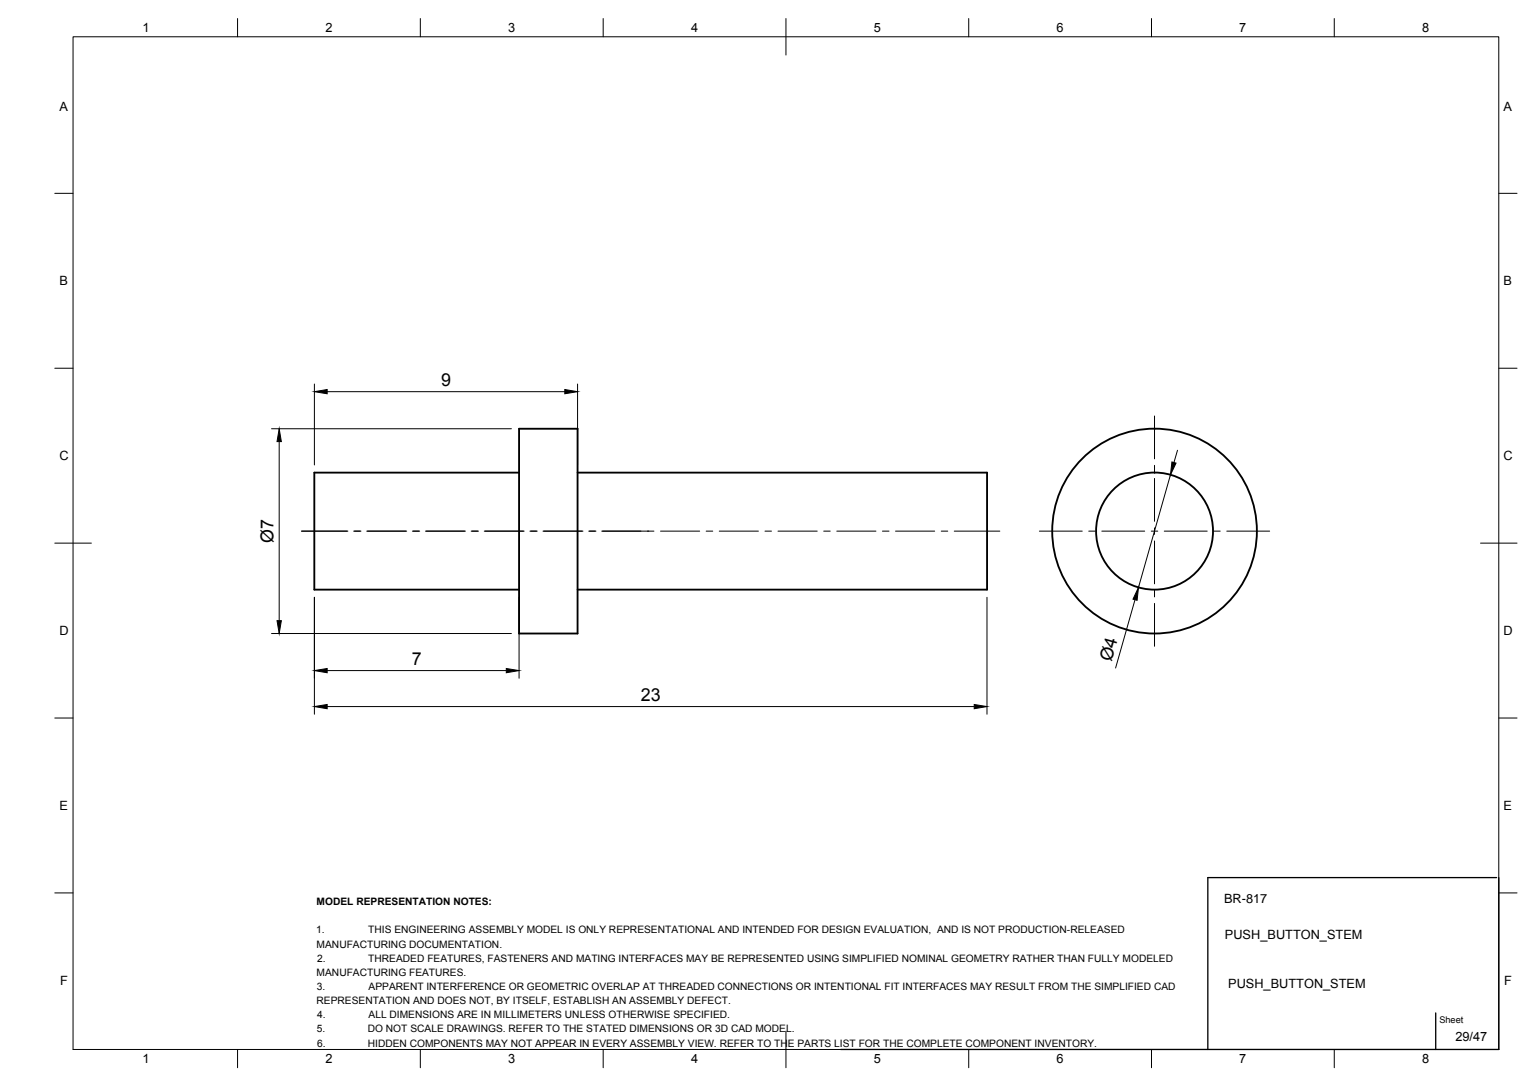
ISO-10303-21;
HEADER;
FILE_DESCRIPTION((''),'2;1');
FILE_NAME('PUSH_BUTTON_STEM.step','2026-10-01T22:07:29-07:00',(''),(''),'','','');
FILE_SCHEMA (('AUTOMOTIVE_DESIGN { 1 0 10303 214 3 1 1 }'));
ENDSEC;
DATA;
#10=MECHANICAL_DESIGN_GEOMETRIC_PRESENTATION_REPRESENTATION('',(#561),#15484);
#491=SHAPE_REPRESENTATION_RELATIONSHIP('SRR','None',#15641,#526) ;
#526=ADVANCED_BREP_SHAPE_REPRESENTATION('',(#602),#15465) ;
#561=STYLED_ITEM('',(#15833),#602) ;
#602=MANIFOLD_SOLID_BREP('PUSH_BUTTON_STEM',#8272) ;
#728=CYLINDRICAL_SURFACE('',#9326,0.35) ;
#729=CYLINDRICAL_SURFACE('',#9327,0.2) ;
#730=CYLINDRICAL_SURFACE('',#9329,0.2) ;
#871=FACE_BOUND('',#2197,.T.) ;
#872=FACE_BOUND('',#2199,.T.) ;
#1139=CIRCLE('',#9321,0.35) ;
#1140=CIRCLE('',#9322,0.2) ;
#1141=CIRCLE('',#9324,0.35) ;
#1142=CIRCLE('',#9325,0.2) ;
#1143=CIRCLE('',#9328,0.2) ;
#1144=CIRCLE('',#9330,0.2) ;
#1635=FACE_OUTER_BOUND('',#2196,.T.) ;
#1636=FACE_OUTER_BOUND('',#2198,.T.) ;
#1637=FACE_OUTER_BOUND('',#2200,.T.) ;
#1638=FACE_OUTER_BOUND('',#2201,.T.) ;
#1639=FACE_OUTER_BOUND('',#2202,.T.) ;
#1640=FACE_OUTER_BOUND('',#2203,.T.) ;
#1641=FACE_OUTER_BOUND('',#2204,.T.) ;
#2196=EDGE_LOOP('',(#6493)) ;
#2197=EDGE_LOOP('',(#6494)) ;
#2198=EDGE_LOOP('',(#6495)) ;
#2199=EDGE_LOOP('',(#6496)) ;
#2200=EDGE_LOOP('',(#6497,#6498,#6499,#6500)) ;
#2201=EDGE_LOOP('',(#6501,#6502,#6503,#6504)) ;
#2202=EDGE_LOOP('',(#6505,#6506,#6507,#6508)) ;
#2203=EDGE_LOOP('',(#6509)) ;
#2204=EDGE_LOOP('',(#6510)) ;
#2719=LINE('',#14264,#3193) ;
#2720=LINE('',#14268,#3194) ;
#2721=LINE('',#14271,#3195) ;
#3193=VECTOR('',#11494,0.35) ;
#3194=VECTOR('',#11499,0.2) ;
#3195=VECTOR('',#11502,0.2) ;
#3795=VERTEX_POINT('',#14254) ;
#3796=VERTEX_POINT('',#14256) ;
#3797=VERTEX_POINT('',#14259) ;
#3798=VERTEX_POINT('',#14261) ;
#3799=VERTEX_POINT('',#14266) ;
#3800=VERTEX_POINT('',#14270) ;
#4751=EDGE_CURVE('',#3795,#3795,#1139,.T.) ;
#4752=EDGE_CURVE('',#3796,#3796,#1140,.T.) ;
#4753=EDGE_CURVE('',#3797,#3797,#1141,.T.) ;
#4754=EDGE_CURVE('',#3798,#3798,#1142,.T.) ;
#4755=EDGE_CURVE('',#3797,#3795,#2719,.T.) ;
#4756=EDGE_CURVE('',#3799,#3799,#1143,.T.) ;
#4757=EDGE_CURVE('',#3799,#3798,#2720,.T.) ;
#4758=EDGE_CURVE('',#3796,#3800,#2721,.T.) ;
#4759=EDGE_CURVE('',#3800,#3800,#1144,.T.) ;
#6493=ORIENTED_EDGE('',*,*,#4751,.T.) ;
#6494=ORIENTED_EDGE('',*,*,#4752,.F.) ;
#6495=ORIENTED_EDGE('',*,*,#4753,.T.) ;
#6496=ORIENTED_EDGE('',*,*,#4754,.F.) ;
#6497=ORIENTED_EDGE('',*,*,#4753,.F.) ;
#6498=ORIENTED_EDGE('',*,*,#4755,.T.) ;
#6499=ORIENTED_EDGE('',*,*,#4751,.F.) ;
#6500=ORIENTED_EDGE('',*,*,#4755,.F.) ;
#6501=ORIENTED_EDGE('',*,*,#4756,.F.) ;
#6502=ORIENTED_EDGE('',*,*,#4757,.T.) ;
#6503=ORIENTED_EDGE('',*,*,#4754,.T.) ;
#6504=ORIENTED_EDGE('',*,*,#4757,.F.) ;
#6505=ORIENTED_EDGE('',*,*,#4752,.T.) ;
#6506=ORIENTED_EDGE('',*,*,#4758,.T.) ;
#6507=ORIENTED_EDGE('',*,*,#4759,.F.) ;
#6508=ORIENTED_EDGE('',*,*,#4758,.F.) ;
#6509=ORIENTED_EDGE('',*,*,#4759,.T.) ;
#6510=ORIENTED_EDGE('',*,*,#4756,.T.) ;
#7660=PLANE('',#9320) ;
#7661=PLANE('',#9323) ;
#7662=PLANE('',#9331) ;
#7663=PLANE('',#9332) ;
#8022=ADVANCED_FACE('',(#1635,#871),#7660,.T.) ;
#8023=ADVANCED_FACE('',(#1636,#872),#7661,.T.) ;
#8024=ADVANCED_FACE('',(#1637),#728,.T.) ;
#8025=ADVANCED_FACE('',(#1638),#729,.T.) ;
#8026=ADVANCED_FACE('',(#1639),#730,.T.) ;
#8027=ADVANCED_FACE('',(#1640),#7662,.T.) ;
#8028=ADVANCED_FACE('',(#1641),#7663,.T.) ;
#8272=CLOSED_SHELL('',(#8022,#8023,#8024,#8025,#8026,#8027,#8028)) ;
#9319=AXIS2_PLACEMENT_3D('',#14252,#11478,#11479) ;
#9320=AXIS2_PLACEMENT_3D('',#14253,#11480,#11481) ;
#9321=AXIS2_PLACEMENT_3D('',#14255,#11482,#11483) ;
#9322=AXIS2_PLACEMENT_3D('',#14257,#11484,#11485) ;
#9323=AXIS2_PLACEMENT_3D('',#14258,#11486,#11487) ;
#9324=AXIS2_PLACEMENT_3D('',#14260,#11488,#11489) ;
#9325=AXIS2_PLACEMENT_3D('',#14262,#11490,#11491) ;
#9326=AXIS2_PLACEMENT_3D('',#14263,#11492,#11493) ;
#9327=AXIS2_PLACEMENT_3D('',#14265,#11495,#11496) ;
#9328=AXIS2_PLACEMENT_3D('',#14267,#11497,#11498) ;
#9329=AXIS2_PLACEMENT_3D('',#14269,#11500,#11501) ;
#9330=AXIS2_PLACEMENT_3D('',#14272,#11503,#11504) ;
#9331=AXIS2_PLACEMENT_3D('',#14273,#11505,#11506) ;
#9332=AXIS2_PLACEMENT_3D('',#14274,#11507,#11508) ;
#11478=DIRECTION('axis',(0.,0.,1.)) ;
#11479=DIRECTION('refdir',(1.,0.,0.)) ;
#11480=DIRECTION('center_axis',(0.,0.,-1.)) ;
#11481=DIRECTION('ref_axis',(-1.,0.,0.)) ;
#11482=DIRECTION('center_axis',(0.,0.,-1.)) ;
#11483=DIRECTION('ref_axis',(1.,0.,0.)) ;
#11484=DIRECTION('center_axis',(0.,0.,-1.)) ;
#11485=DIRECTION('ref_axis',(1.,0.,0.)) ;
#11486=DIRECTION('center_axis',(0.,0.,1.)) ;
#11487=DIRECTION('ref_axis',(1.,0.,0.)) ;
#11488=DIRECTION('center_axis',(0.,0.,1.)) ;
#11489=DIRECTION('ref_axis',(1.,0.,0.)) ;
#11490=DIRECTION('center_axis',(0.,0.,1.)) ;
#11491=DIRECTION('ref_axis',(1.,0.,0.)) ;
#11492=DIRECTION('center_axis',(0.,0.,1.)) ;
#11493=DIRECTION('ref_axis',(1.,0.,0.)) ;
#11494=DIRECTION('',(0.,0.,-1.)) ;
#11495=DIRECTION('center_axis',(0.,0.,1.)) ;
#11496=DIRECTION('ref_axis',(1.,0.,0.)) ;
#11497=DIRECTION('center_axis',(0.,0.,1.)) ;
#11498=DIRECTION('ref_axis',(1.,0.,0.)) ;
#11499=DIRECTION('',(0.,0.,-1.)) ;
#11500=DIRECTION('center_axis',(0.,0.,1.)) ;
#11501=DIRECTION('ref_axis',(1.,0.,0.)) ;
#11502=DIRECTION('',(0.,0.,-1.)) ;
#11503=DIRECTION('center_axis',(0.,0.,-1.)) ;
#11504=DIRECTION('ref_axis',(1.,0.,0.)) ;
#11505=DIRECTION('center_axis',(0.,0.,-1.)) ;
#11506=DIRECTION('ref_axis',(-1.,0.,0.)) ;
#11507=DIRECTION('center_axis',(0.,0.,1.)) ;
#11508=DIRECTION('ref_axis',(1.,0.,0.)) ;
#14252=CARTESIAN_POINT('',(0.,0.,0.)) ;
#14253=CARTESIAN_POINT('Origin',(-3.,1.8,1.7)) ;
#14254=CARTESIAN_POINT('',(-3.35,1.8,1.7)) ;
#14255=CARTESIAN_POINT('Origin',(-3.,1.8,1.7)) ;
#14256=CARTESIAN_POINT('',(-3.2,1.8,1.7)) ;
#14257=CARTESIAN_POINT('Origin',(-3.,1.8,1.7)) ;
#14258=CARTESIAN_POINT('Origin',(-3.,1.8,1.9)) ;
#14259=CARTESIAN_POINT('',(-3.35,1.8,1.9)) ;
#14260=CARTESIAN_POINT('Origin',(-3.,1.8,1.9)) ;
#14261=CARTESIAN_POINT('',(-3.2,1.8,1.9)) ;
#14262=CARTESIAN_POINT('Origin',(-3.,1.8,1.9)) ;
#14263=CARTESIAN_POINT('Origin',(-3.,1.8,1.8)) ;
#14264=CARTESIAN_POINT('',(-3.35,1.8,1.8)) ;
#14265=CARTESIAN_POINT('Origin',(-3.,1.8,1.45)) ;
#14266=CARTESIAN_POINT('',(-3.2,1.8,2.6)) ;
#14267=CARTESIAN_POINT('Origin',(-3.,1.8,2.6)) ;
#14268=CARTESIAN_POINT('',(-3.2,1.8,1.45)) ;
#14269=CARTESIAN_POINT('Origin',(-3.,1.8,1.45)) ;
#14270=CARTESIAN_POINT('',(-3.2,1.8,0.3)) ;
#14271=CARTESIAN_POINT('',(-3.2,1.8,1.45)) ;
#14272=CARTESIAN_POINT('Origin',(-3.,1.8,0.3)) ;
#14273=CARTESIAN_POINT('Origin',(-3.,1.8,0.3)) ;
#14274=CARTESIAN_POINT('Origin',(-3.,1.8,2.6)) ;
#15422=UNCERTAINTY_MEASURE_WITH_UNIT(LENGTH_MEASURE(0.001),#15485,
'DISTANCE_ACCURACY_VALUE',
'Maximum model space distance between geometric entities at asserted c
onnectivities') ;
#15441=UNCERTAINTY_MEASURE_WITH_UNIT(LENGTH_MEASURE(0.001),#15485,
'DISTANCE_ACCURACY_VALUE',
'Maximum model space distance between geometric entities at asserted c
onnectivities') ;
#15465=(
GEOMETRIC_REPRESENTATION_CONTEXT(3)
GLOBAL_UNCERTAINTY_ASSIGNED_CONTEXT((#15422))
GLOBAL_UNIT_ASSIGNED_CONTEXT((#15485,#15487,#15488))
REPRESENTATION_CONTEXT('','3D')
) ;
#15484=(
GEOMETRIC_REPRESENTATION_CONTEXT(3)
GLOBAL_UNCERTAINTY_ASSIGNED_CONTEXT((#15441))
GLOBAL_UNIT_ASSIGNED_CONTEXT((#15485,#15487,#15488))
REPRESENTATION_CONTEXT('','3D')
) ;
#15485=(
LENGTH_UNIT()
NAMED_UNIT(*)
SI_UNIT(.CENTI.,.METRE.)
) ;
#15487=(
NAMED_UNIT(*)
PLANE_ANGLE_UNIT()
SI_UNIT($,.RADIAN.)
) ;
#15488=(
NAMED_UNIT(*)
SI_UNIT($,.STERADIAN.)
SOLID_ANGLE_UNIT()
) ;
#15512=SHAPE_DEFINITION_REPRESENTATION(#15569,#15641) ;
#15569=PRODUCT_DEFINITION_SHAPE('',$,#15684) ;
#15641=SHAPE_REPRESENTATION('',(#9319),#15465) ;
#15660=PRODUCT_DEFINITION_CONTEXT('part definition',#15788,'design') ;
#15684=PRODUCT_DEFINITION('PUSH_BUTTON_STEM','PUSH_BUTTON_STEM',
#15726,#15660) ;
#15726=PRODUCT_DEFINITION_FORMATION('',$,#15813) ;
#15788=APPLICATION_CONTEXT(
'Core Data for Automotive Mechanical Design Process') ;
#15789=PRODUCT_CONTEXT('part definition',#15788,'mechanical') ;
#15813=PRODUCT('PUSH_BUTTON_STEM','PUSH_BUTTON_STEM',$,(#15789)) ;
#15833=PRESENTATION_STYLE_ASSIGNMENT((#15845)) ;
#15845=SURFACE_STYLE_USAGE(.BOTH.,#15857) ;
#15857=SURFACE_SIDE_STYLE('',(#15869)) ;
#15869=SURFACE_STYLE_FILL_AREA(#15881) ;
#15881=FILL_AREA_STYLE('Nylon 6-6 (White)',(#15893)) ;
#15893=FILL_AREA_STYLE_COLOUR('Nylon 6-6 (White)',#15905) ;
#15905=COLOUR_RGB('Nylon 6-6 (White)', 0.31764706, 0.68627451, 0.89019608) ;
ENDSEC;
END-ISO-10303-21;
